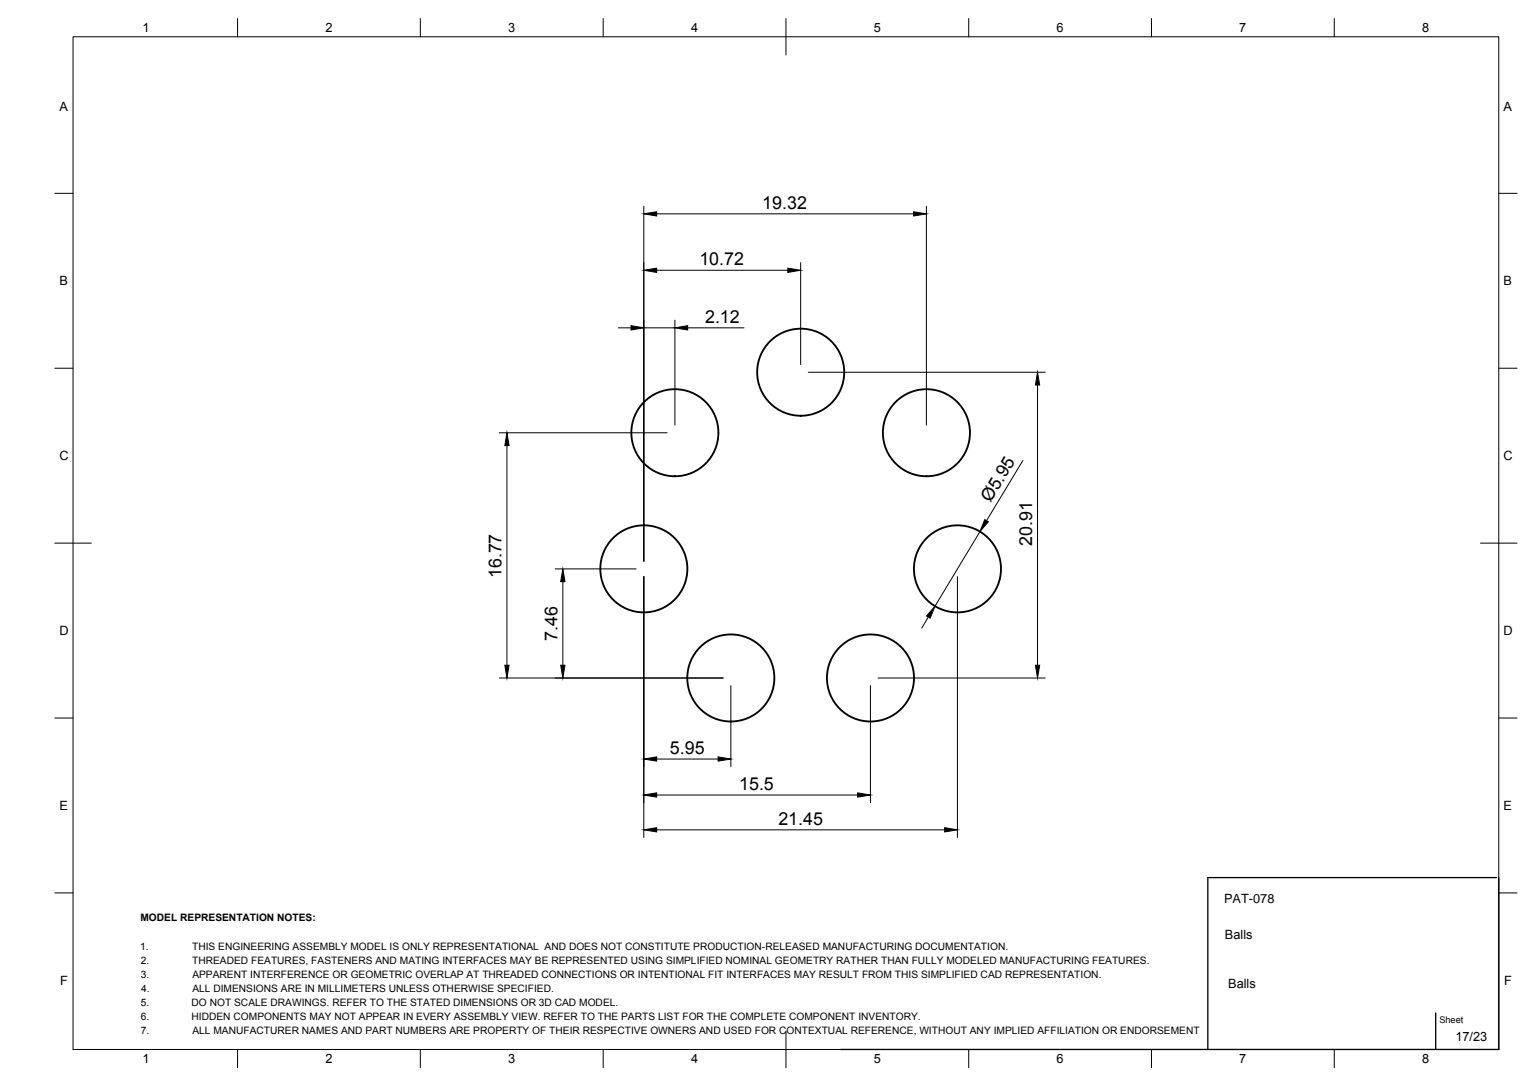
ISO-10303-21;
HEADER;
/* Generated by software containing ST-Developer
 * from STEP Tools, Inc. (www.steptools.com) 
 */

FILE_DESCRIPTION(
/* description */ ('Pedal-braked fixed caster'),
/* implementation_level */ '2;1');

FILE_NAME(
/* name */ 'Balls.step',
/* time_stamp */ '2026-10-28T03:26:52-07:00',
/* author */ (''),
/* organization */ (''),
/* preprocessor_version */ 'ST-DEVELOPER v20.2',
/* originating_system */ 'Autodesk Translation Framework v15.17.0.0',
/* authorisation */ '');

FILE_SCHEMA (('AUTOMOTIVE_DESIGN { 1 0 10303 214 3 1 1 }'));
ENDSEC;

DATA;
#10=MECHANICAL_DESIGN_GEOMETRIC_PRESENTATION_REPRESENTATION('',(#217,#218,#219,#220,#221,#222,#223),#5734);
#25=SPHERICAL_SURFACE('',#3429,0.29765);
#26=SPHERICAL_SURFACE('',#3431,0.29765);
#27=SPHERICAL_SURFACE('',#3433,0.29765);
#28=SPHERICAL_SURFACE('',#3435,0.29765);
#29=SPHERICAL_SURFACE('',#3437,0.29765);
#30=SPHERICAL_SURFACE('',#3439,0.29765);
#31=SPHERICAL_SURFACE('',#3441,0.29765);
#183=SHAPE_REPRESENTATION_RELATIONSHIP('SRR','None',#5823,#200);
#200=ADVANCED_BREP_SHAPE_REPRESENTATION('',(#240,#241,#242,#243,#244,#245,
#246),#5727);
#217=STYLED_ITEM('',(#5984),#240);
#218=STYLED_ITEM('',(#5984),#241);
#219=STYLED_ITEM('',(#5984),#242);
#220=STYLED_ITEM('',(#5984),#243);
#221=STYLED_ITEM('',(#5984),#244);
#222=STYLED_ITEM('',(#5984),#245);
#223=STYLED_ITEM('',(#5984),#246);
#240=MANIFOLD_SOLID_BREP('Body1',#2999);
#241=MANIFOLD_SOLID_BREP('Body2',#3000);
#242=MANIFOLD_SOLID_BREP('Body3',#3001);
#243=MANIFOLD_SOLID_BREP('Body4',#3002);
#244=MANIFOLD_SOLID_BREP('Body5',#3003);
#245=MANIFOLD_SOLID_BREP('Body6',#3004);
#246=MANIFOLD_SOLID_BREP('Body7',#3005);
#419=CIRCLE('',#3430,0.29765);
#420=CIRCLE('',#3432,0.29765);
#421=CIRCLE('',#3434,0.29765);
#422=CIRCLE('',#3436,0.29765);
#423=CIRCLE('',#3438,0.29765);
#424=CIRCLE('',#3440,0.29765);
#425=CIRCLE('',#3442,0.29765);
#600=FACE_OUTER_BOUND('',#814,.T.);
#601=FACE_OUTER_BOUND('',#815,.T.);
#602=FACE_OUTER_BOUND('',#816,.T.);
#603=FACE_OUTER_BOUND('',#817,.T.);
#604=FACE_OUTER_BOUND('',#818,.T.);
#605=FACE_OUTER_BOUND('',#819,.T.);
#606=FACE_OUTER_BOUND('',#820,.T.);
#814=EDGE_LOOP('',(#2470,#2471));
#815=EDGE_LOOP('',(#2472,#2473));
#816=EDGE_LOOP('',(#2474,#2475));
#817=EDGE_LOOP('',(#2476,#2477));
#818=EDGE_LOOP('',(#2478,#2479));
#819=EDGE_LOOP('',(#2480,#2481));
#820=EDGE_LOOP('',(#2482,#2483));
#1474=VERTEX_POINT('',#5120);
#1475=VERTEX_POINT('',#5121);
#1476=VERTEX_POINT('',#5124);
#1477=VERTEX_POINT('',#5125);
#1478=VERTEX_POINT('',#5128);
#1479=VERTEX_POINT('',#5129);
#1480=VERTEX_POINT('',#5132);
#1481=VERTEX_POINT('',#5133);
#1482=VERTEX_POINT('',#5136);
#1483=VERTEX_POINT('',#5137);
#1484=VERTEX_POINT('',#5140);
#1485=VERTEX_POINT('',#5141);
#1486=VERTEX_POINT('',#5144);
#1487=VERTEX_POINT('',#5145);
#1825=EDGE_CURVE('',#1474,#1475,#419,.T.);
#1826=EDGE_CURVE('',#1476,#1477,#420,.T.);
#1827=EDGE_CURVE('',#1478,#1479,#421,.T.);
#1828=EDGE_CURVE('',#1480,#1481,#422,.T.);
#1829=EDGE_CURVE('',#1482,#1483,#423,.T.);
#1830=EDGE_CURVE('',#1484,#1485,#424,.T.);
#1831=EDGE_CURVE('',#1486,#1487,#425,.T.);
#2470=ORIENTED_EDGE('',*,*,#1825,.T.);
#2471=ORIENTED_EDGE('',*,*,#1825,.F.);
#2472=ORIENTED_EDGE('',*,*,#1826,.T.);
#2473=ORIENTED_EDGE('',*,*,#1826,.F.);
#2474=ORIENTED_EDGE('',*,*,#1827,.T.);
#2475=ORIENTED_EDGE('',*,*,#1827,.F.);
#2476=ORIENTED_EDGE('',*,*,#1828,.T.);
#2477=ORIENTED_EDGE('',*,*,#1828,.F.);
#2478=ORIENTED_EDGE('',*,*,#1829,.T.);
#2479=ORIENTED_EDGE('',*,*,#1829,.F.);
#2480=ORIENTED_EDGE('',*,*,#1830,.T.);
#2481=ORIENTED_EDGE('',*,*,#1830,.F.);
#2482=ORIENTED_EDGE('',*,*,#1831,.T.);
#2483=ORIENTED_EDGE('',*,*,#1831,.F.);
#2933=ADVANCED_FACE('',(#600),#25,.T.);
#2934=ADVANCED_FACE('',(#601),#26,.T.);
#2935=ADVANCED_FACE('',(#602),#27,.T.);
#2936=ADVANCED_FACE('',(#603),#28,.T.);
#2937=ADVANCED_FACE('',(#604),#29,.T.);
#2938=ADVANCED_FACE('',(#605),#30,.T.);
#2939=ADVANCED_FACE('',(#606),#31,.T.);
#2999=CLOSED_SHELL('',(#2933));
#3000=CLOSED_SHELL('',(#2934));
#3001=CLOSED_SHELL('',(#2935));
#3002=CLOSED_SHELL('',(#2936));
#3003=CLOSED_SHELL('',(#2937));
#3004=CLOSED_SHELL('',(#2938));
#3005=CLOSED_SHELL('',(#2939));
#3428=AXIS2_PLACEMENT_3D('',#5118,#4185,#4186);
#3429=AXIS2_PLACEMENT_3D('',#5119,#4187,#4188);
#3430=AXIS2_PLACEMENT_3D('',#5122,#4189,#4190);
#3431=AXIS2_PLACEMENT_3D('',#5123,#4191,#4192);
#3432=AXIS2_PLACEMENT_3D('',#5126,#4193,#4194);
#3433=AXIS2_PLACEMENT_3D('',#5127,#4195,#4196);
#3434=AXIS2_PLACEMENT_3D('',#5130,#4197,#4198);
#3435=AXIS2_PLACEMENT_3D('',#5131,#4199,#4200);
#3436=AXIS2_PLACEMENT_3D('',#5134,#4201,#4202);
#3437=AXIS2_PLACEMENT_3D('',#5135,#4203,#4204);
#3438=AXIS2_PLACEMENT_3D('',#5138,#4205,#4206);
#3439=AXIS2_PLACEMENT_3D('',#5139,#4207,#4208);
#3440=AXIS2_PLACEMENT_3D('',#5142,#4209,#4210);
#3441=AXIS2_PLACEMENT_3D('',#5143,#4211,#4212);
#3442=AXIS2_PLACEMENT_3D('',#5146,#4213,#4214);
#4185=DIRECTION('axis',(0.,0.,1.));
#4186=DIRECTION('refdir',(1.,0.,0.));
#4187=DIRECTION('center_axis',(0.,0.,1.));
#4188=DIRECTION('ref_axis',(1.,0.,0.));
#4189=DIRECTION('center_axis',(1.22464679914735E-16,-1.,0.));
#4190=DIRECTION('ref_axis',(-1.,-1.22464679914735E-16,0.));
#4191=DIRECTION('center_axis',(0.78183148246803,0.,0.623489801858733));
#4192=DIRECTION('ref_axis',(0.623489801858734,0.,-0.78183148246803));
#4193=DIRECTION('center_axis',(7.63554790147315E-17,-1.,-9.57467422477103E-17));
#4194=DIRECTION('ref_axis',(-0.623489801858734,-1.22464679914735E-16,0.78183148246803));
#4195=DIRECTION('center_axis',(0.974927912181824,0.,-0.222520933956314));
#4196=DIRECTION('ref_axis',(-0.222520933956314,0.,-0.974927912181824));
#4197=DIRECTION('center_axis',(-2.7250954951288E-17,-1.,-1.19394234705288E-16));
#4198=DIRECTION('ref_axis',(0.222520933956314,-1.22464679914735E-16,0.974927912181824));
#4199=DIRECTION('center_axis',(0.433883739117558,0.,-0.900968867902419));
#4200=DIRECTION('ref_axis',(-0.900968867902419,0.,-0.433883739117558));
#4201=DIRECTION('center_axis',(-1.10336864020811E-16,-1.,-5.31354332312403E-17));
#4202=DIRECTION('ref_axis',(0.900968867902419,-1.22464679914735E-16,0.433883739117558));
#4203=DIRECTION('center_axis',(-0.433883739117558,0.,-0.900968867902419));
#4204=DIRECTION('ref_axis',(-0.900968867902419,0.,0.433883739117558));
#4205=DIRECTION('center_axis',(-1.10336864020811E-16,-1.,5.31354332312403E-17));
#4206=DIRECTION('ref_axis',(0.900968867902419,-1.22464679914735E-16,-0.433883739117558));
#4207=DIRECTION('center_axis',(-0.974927912181824,0.,-0.222520933956314));
#4208=DIRECTION('ref_axis',(-0.222520933956315,0.,0.974927912181824));
#4209=DIRECTION('center_axis',(-2.7250954951288E-17,-1.,1.19394234705288E-16));
#4210=DIRECTION('ref_axis',(0.222520933956315,-1.22464679914735E-16,-0.974927912181824));
#4211=DIRECTION('center_axis',(-0.78183148246803,0.,0.623489801858734));
#4212=DIRECTION('ref_axis',(0.623489801858733,0.,0.78183148246803));
#4213=DIRECTION('center_axis',(7.63554790147315E-17,-1.,9.57467422477103E-17));
#4214=DIRECTION('ref_axis',(-0.623489801858733,-1.22464679914735E-16,-0.78183148246803));
#5118=CARTESIAN_POINT('',(0.,0.,0.));
#5119=CARTESIAN_POINT('Origin',(1.1,0.,0.));
#5120=CARTESIAN_POINT('',(1.1,-2.23201749654651E-33,0.29765));
#5121=CARTESIAN_POINT('',(1.1,-2.23201749654651E-33,-0.29765));
#5122=CARTESIAN_POINT('Origin',(1.1,0.,0.));
#5123=CARTESIAN_POINT('Origin',(0.685838782044607,0.,-0.860014630714833));
#5124=CARTESIAN_POINT('',(0.918550922801216,-5.31350540756609E-33,-0.674432891191581));
#5125=CARTESIAN_POINT('',(0.453126641287998,8.49470414473068E-34,-1.04559637023808));
#5126=CARTESIAN_POINT('Origin',(0.685838782044607,0.,-0.860014630714833));
#5127=CARTESIAN_POINT('Origin',(-0.244773027351946,0.,-1.07242070340001));
#5128=CARTESIAN_POINT('',(0.0454142657089739,-2.23201749654651E-33,-1.1386540593921));
#5129=CARTESIAN_POINT('',(-0.534960320412865,-2.23201749654651E-33,-1.00618734740791));
#5130=CARTESIAN_POINT('Origin',(-0.244773027351946,0.,-1.07242070340001));
#5131=CARTESIAN_POINT('Origin',(-0.991065754692661,0.,-0.477272113029314));
#5132=CARTESIAN_POINT('',(-0.86192025974432,8.49470414473067E-34,-0.745445496560469));
#5133=CARTESIAN_POINT('',(-1.120211249641,-5.31350540756609E-33,-0.209098729498159));
#5134=CARTESIAN_POINT('Origin',(-0.991065754692661,0.,-0.477272113029314));
#5135=CARTESIAN_POINT('Origin',(-0.991065754692661,0.,0.477272113029314));
#5136=CARTESIAN_POINT('',(-1.120211249641,-2.23201749654651E-33,0.209098729498159));
#5137=CARTESIAN_POINT('',(-0.86192025974432,-2.23201749654651E-33,0.745445496560469));
#5138=CARTESIAN_POINT('Origin',(-0.991065754692661,0.,0.477272113029314));
#5139=CARTESIAN_POINT('Origin',(-0.244773027351946,0.,1.07242070340001));
#5140=CARTESIAN_POINT('',(-0.534960320412866,-2.23201749654651E-33,1.00618734740791));
#5141=CARTESIAN_POINT('',(0.0454142657089737,-2.23201749654651E-33,1.1386540593921));
#5142=CARTESIAN_POINT('Origin',(-0.244773027351946,0.,1.07242070340001));
#5143=CARTESIAN_POINT('Origin',(0.685838782044607,0.,0.860014630714833));
#5144=CARTESIAN_POINT('',(0.453126641287998,-2.23201749654651E-33,1.04559637023808));
#5145=CARTESIAN_POINT('',(0.918550922801216,-2.23201749654651E-33,0.674432891191581));
#5146=CARTESIAN_POINT('Origin',(0.685838782044607,0.,0.860014630714833));
#5704=UNCERTAINTY_MEASURE_WITH_UNIT(LENGTH_MEASURE(0.001),#5735,
'DISTANCE_ACCURACY_VALUE',
'Maximum model space distance between geometric entities at asserted c
onnectivities');
#5711=UNCERTAINTY_MEASURE_WITH_UNIT(LENGTH_MEASURE(0.001),#5735,
'DISTANCE_ACCURACY_VALUE',
'Maximum model space distance between geometric entities at asserted c
onnectivities');
#5727=(
GEOMETRIC_REPRESENTATION_CONTEXT(3)
GLOBAL_UNCERTAINTY_ASSIGNED_CONTEXT((#5704))
GLOBAL_UNIT_ASSIGNED_CONTEXT((#5735,#5737,#5738))
REPRESENTATION_CONTEXT('','3D')
);
#5734=(
GEOMETRIC_REPRESENTATION_CONTEXT(3)
GLOBAL_UNCERTAINTY_ASSIGNED_CONTEXT((#5711))
GLOBAL_UNIT_ASSIGNED_CONTEXT((#5735,#5737,#5738))
REPRESENTATION_CONTEXT('','3D')
);
#5735=(
LENGTH_UNIT()
NAMED_UNIT(*)
SI_UNIT(.CENTI.,.METRE.)
);
#5737=(
NAMED_UNIT(*)
PLANE_ANGLE_UNIT()
SI_UNIT($,.RADIAN.)
);
#5738=(
NAMED_UNIT(*)
SI_UNIT($,.STERADIAN.)
SOLID_ANGLE_UNIT()
);
#5754=SHAPE_DEFINITION_REPRESENTATION(#5786,#5823);
#5786=PRODUCT_DEFINITION_SHAPE('',$,#5846);
#5823=SHAPE_REPRESENTATION('',(#3428),#5727);
#5830=PRODUCT_DEFINITION_CONTEXT('part definition',#5898,'design');
#5846=PRODUCT_DEFINITION('Balls','Balls',#5868,#5830);
#5868=PRODUCT_DEFINITION_FORMATION('',$,#5915);
#5898=APPLICATION_CONTEXT(
'Core Data for Automotive Mechanical Design Process');
#5899=PRODUCT_CONTEXT('part definition',#5898,'mechanical');
#5915=PRODUCT('Balls','Balls','Balls',(#5899));
#5978=COLOUR_RGB('Grey',0.48,0.52,0.57);
#5979=FILL_AREA_STYLE_COLOUR('',#5978);
#5980=FILL_AREA_STYLE('',(#5979));
#5981=SURFACE_STYLE_FILL_AREA(#5980);
#5982=SURFACE_SIDE_STYLE('',(#5981));
#5983=SURFACE_STYLE_USAGE(.BOTH.,#5982);
#5984=PRESENTATION_STYLE_ASSIGNMENT((#5983));
ENDSEC;
END-ISO-10303-21;
